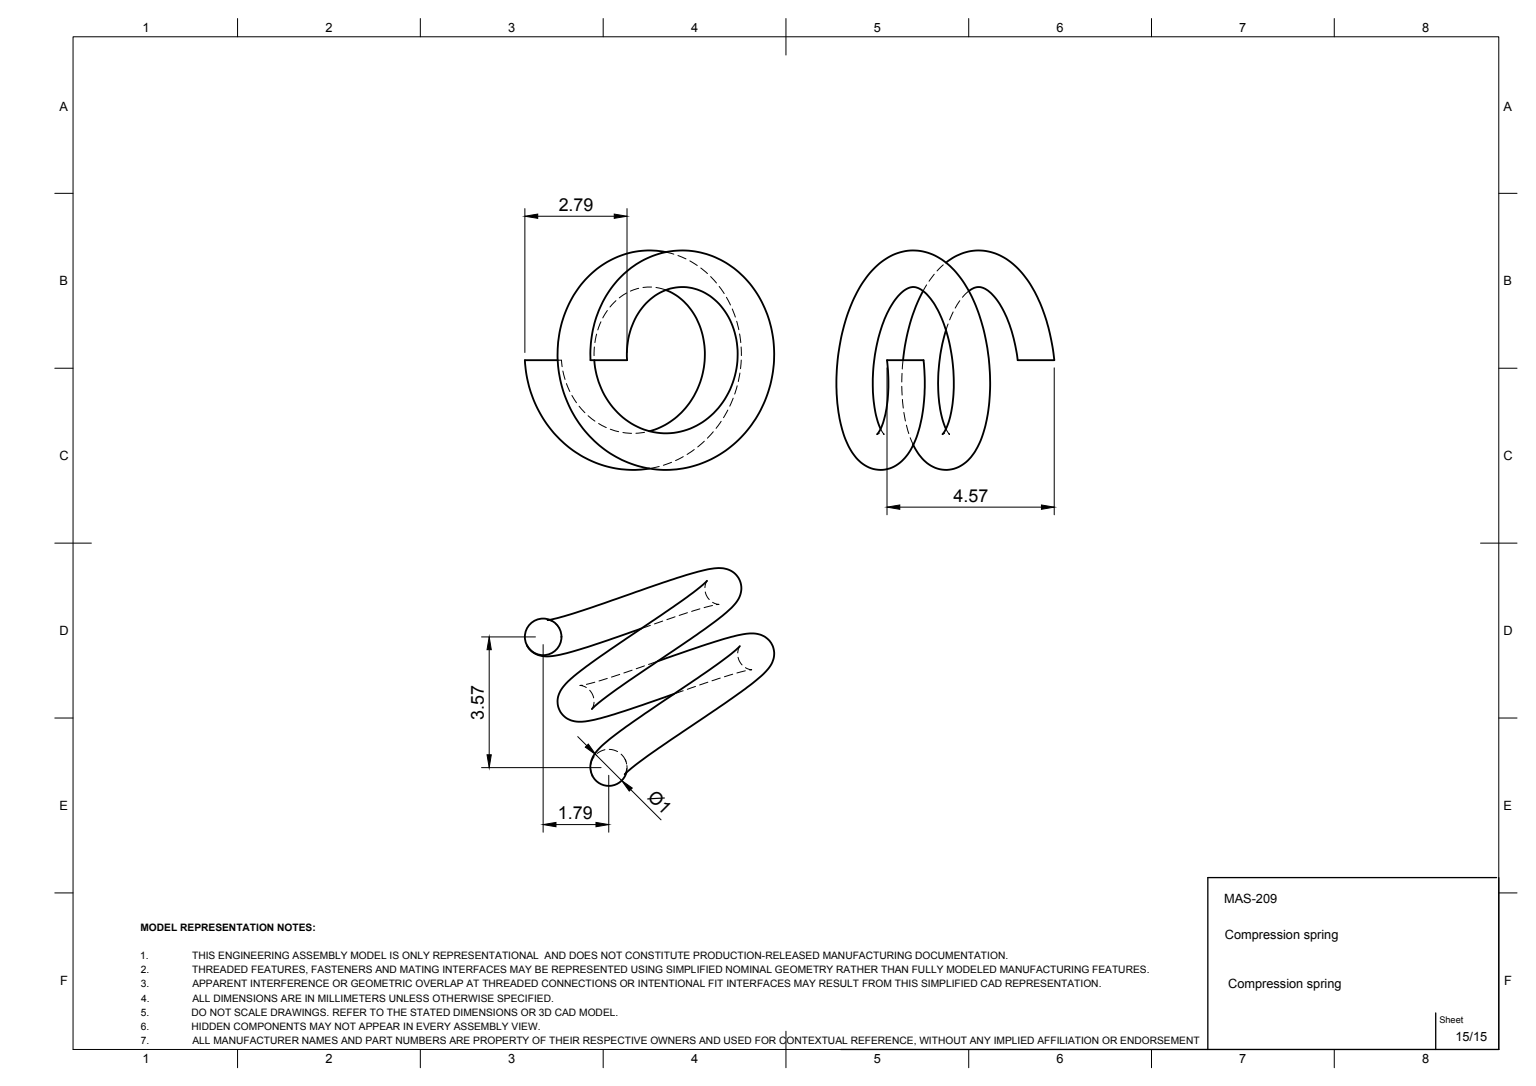
ISO-10303-21;
HEADER;
/* Generated by software containing ST-Developer
 * from STEP Tools, Inc. (www.steptools.com) 
 */

FILE_DESCRIPTION(
/* description */ ('Independent bearing-supported roller-ramp one-way clutch. Six logarit
hmic ramps with plain solid rollers, sprung guided plungers, native Co
il variants, removable shared keepers, rounded parallel key, shaft wit
h complete retaining lips, bronze journal/thrust support and bolted co
vers. Native rotor, roller planar/spin and plunger joints permit manua
l geometric engaged/released inspection. Automatic frictional torque s
witching/contact dynamics are not simulated; no capacity, hardness, fi
t, lubrication, speed, force or life rating. External input driver/cou
pling/anchors outside assembly.'),
/* implementation_level */ '2;1');

FILE_NAME(
/* name */ 'Compression spring.step',
/* time_stamp */ '2026-11-08T07:04:38-08:00',
/* author */ (''),
/* organization */ (''),
/* preprocessor_version */ 'ST-DEVELOPER v20.2',
/* originating_system */ 'Autodesk Translation Framework v15.17.0.0',
/* authorisation */ '');

FILE_SCHEMA (('AUTOMOTIVE_DESIGN { 1 0 10303 214 3 1 1 }'));
ENDSEC;

DATA;
#10=MECHANICAL_DESIGN_GEOMETRIC_PRESENTATION_REPRESENTATION('',(#313),#99526);
#281=SHAPE_REPRESENTATION_RELATIONSHIP('SRR','None',#99638,#297);
#297=ADVANCED_BREP_SHAPE_REPRESENTATION('',(#329),#99523);
#313=STYLED_ITEM('',(#99724),#329);
#329=MANIFOLD_SOLID_BREP('Body1',#18283);
#592=PLANE('',#19645);
#593=PLANE('',#19646);
#670=B_SPLINE_SURFACE_WITH_KNOTS('',3,3,((#94938,#94939,#94940,#94941,#94942,
#94943,#94944,#94945,#94946,#94947,#94948,#94949,#94950,#94951,#94952,#94953,
#94954,#94955,#94956,#94957,#94958,#94959,#94960,#94961,#94962,#94963,#94964,
#94965,#94966),(#94967,#94968,#94969,#94970,#94971,#94972,#94973,#94974,
#94975,#94976,#94977,#94978,#94979,#94980,#94981,#94982,#94983,#94984,#94985,
#94986,#94987,#94988,#94989,#94990,#94991,#94992,#94993,#94994,#94995),
(#94996,#94997,#94998,#94999,#95000,#95001,#95002,#95003,#95004,#95005,
#95006,#95007,#95008,#95009,#95010,#95011,#95012,#95013,#95014,#95015,#95016,
#95017,#95018,#95019,#95020,#95021,#95022,#95023,#95024),(#95025,#95026,
#95027,#95028,#95029,#95030,#95031,#95032,#95033,#95034,#95035,#95036,#95037,
#95038,#95039,#95040,#95041,#95042,#95043,#95044,#95045,#95046,#95047,#95048,
#95049,#95050,#95051,#95052,#95053),(#95054,#95055,#95056,#95057,#95058,
#95059,#95060,#95061,#95062,#95063,#95064,#95065,#95066,#95067,#95068,#95069,
#95070,#95071,#95072,#95073,#95074,#95075,#95076,#95077,#95078,#95079,#95080,
#95081,#95082),(#95083,#95084,#95085,#95086,#95087,#95088,#95089,#95090,
#95091,#95092,#95093,#95094,#95095,#95096,#95097,#95098,#95099,#95100,#95101,
#95102,#95103,#95104,#95105,#95106,#95107,#95108,#95109,#95110,#95111),
(#95112,#95113,#95114,#95115,#95116,#95117,#95118,#95119,#95120,#95121,
#95122,#95123,#95124,#95125,#95126,#95127,#95128,#95129,#95130,#95131,#95132,
#95133,#95134,#95135,#95136,#95137,#95138,#95139,#95140),(#95141,#95142,
#95143,#95144,#95145,#95146,#95147,#95148,#95149,#95150,#95151,#95152,#95153,
#95154,#95155,#95156,#95157,#95158,#95159,#95160,#95161,#95162,#95163,#95164,
#95165,#95166,#95167,#95168,#95169),(#95170,#95171,#95172,#95173,#95174,
#95175,#95176,#95177,#95178,#95179,#95180,#95181,#95182,#95183,#95184,#95185,
#95186,#95187,#95188,#95189,#95190,#95191,#95192,#95193,#95194,#95195,#95196,
#95197,#95198),(#95199,#95200,#95201,#95202,#95203,#95204,#95205,#95206,
#95207,#95208,#95209,#95210,#95211,#95212,#95213,#95214,#95215,#95216,#95217,
#95218,#95219,#95220,#95221,#95222,#95223,#95224,#95225,#95226,#95227)),
 .UNSPECIFIED.,.T.,.F.,.F.,(4,1,1,1,1,1,1,4),(4,1,1,1,1,1,1,1,1,1,1,1,1,
1,1,1,1,1,1,1,1,1,1,1,1,1,4),(-3.14159265358979,-2.24399475256414,-1.34639685153848,
-0.448798950512828,0.448798950512828,1.34639685153848,2.24399475256414,
3.14159265358979),(0.,0.483321946706122,0.966643893412244,1.44996584011837,
1.93328778682449,2.41660973353061,2.89993168023673,3.38325362694285,3.86657557364898,
4.3498975203551,4.83321946706122,5.31654141376734,5.79986336047346,6.28318530717959,
6.76650725388571,7.24982920059183,7.73315114729795,8.21647309400407,8.6997950407102,
9.18311698741632,9.66643893412244,10.1497608808286,10.6330828275347,11.1164047742408,
11.5997267209469,12.083048667653,12.5663706143592),.UNSPECIFIED.);
#1589=FACE_OUTER_BOUND('',#2691,.T.);
#1590=FACE_OUTER_BOUND('',#2692,.T.);
#1591=FACE_OUTER_BOUND('',#2693,.T.);
#2691=EDGE_LOOP('',(#16092,#16093,#16094,#16095));
#2692=EDGE_LOOP('',(#16096));
#2693=EDGE_LOOP('',(#16097));
#3096=CIRCLE('',#19643,0.5);
#3097=CIRCLE('',#19644,0.5);
#4515=B_SPLINE_CURVE_WITH_KNOTS('',3,(#95231,#95232,#95233,#95234,#95235,
#95236,#95237,#95238,#95239,#95240,#95241,#95242,#95243,#95244,#95245,#95246,
#95247,#95248,#95249,#95250,#95251,#95252,#95253,#95254,#95255,#95256,#95257,
#95258,#95259),.UNSPECIFIED.,.F.,.F.,(4,1,1,1,1,1,1,1,1,1,1,1,1,1,1,1,1,
1,1,1,1,1,1,1,1,1,4),(0.,0.483321946706122,0.966643893412244,1.44996584011837,
1.93328778682449,2.41660973353061,2.89993168023673,3.38325362694285,3.86657557364898,
4.3498975203551,4.83321946706122,5.31654141376734,5.79986336047346,6.28318530717959,
6.76650725388571,7.24982920059183,7.73315114729795,8.21647309400407,8.6997950407102,
9.18311698741632,9.66643893412244,10.1497608808286,10.6330828275347,11.1164047742408,
11.5997267209469,12.083048667653,12.5663706143592),.UNSPECIFIED.);
#8115=VERTEX_POINT('',#95228);
#8116=VERTEX_POINT('',#95230);
#10798=EDGE_CURVE('',#8115,#8115,#3096,.T.);
#10799=EDGE_CURVE('',#8115,#8116,#4515,.T.);
#10800=EDGE_CURVE('',#8116,#8116,#3097,.T.);
#16092=ORIENTED_EDGE('',*,*,#10798,.T.);
#16093=ORIENTED_EDGE('',*,*,#10799,.T.);
#16094=ORIENTED_EDGE('',*,*,#10800,.F.);
#16095=ORIENTED_EDGE('',*,*,#10799,.F.);
#16096=ORIENTED_EDGE('',*,*,#10800,.T.);
#16097=ORIENTED_EDGE('',*,*,#10798,.F.);
#18187=ADVANCED_FACE('',(#1589),#670,.T.);
#18188=ADVANCED_FACE('',(#1590),#592,.F.);
#18189=ADVANCED_FACE('',(#1591),#593,.T.);
#18283=CLOSED_SHELL('',(#18187,#18188,#18189));
#19642=AXIS2_PLACEMENT_3D('',#94937,#22973,#22974);
#19643=AXIS2_PLACEMENT_3D('',#95229,#22975,#22976);
#19644=AXIS2_PLACEMENT_3D('',#95260,#22977,#22978);
#19645=AXIS2_PLACEMENT_3D('',#95261,#22979,#22980);
#19646=AXIS2_PLACEMENT_3D('',#95262,#22981,#22982);
#22973=DIRECTION('axis',(0.,0.,1.));
#22974=DIRECTION('refdir',(1.,0.,0.));
#22975=DIRECTION('center_axis',(0.,0.,-1.));
#22976=DIRECTION('ref_axis',(-1.,0.,0.));
#22977=DIRECTION('center_axis',(4.89858719658941E-16,0.,-1.));
#22978=DIRECTION('ref_axis',(-1.,0.,-4.89858719658941E-16));
#22979=DIRECTION('center_axis',(-4.89858719658941E-16,0.,1.));
#22980=DIRECTION('ref_axis',(1.,0.,4.89858719658941E-16));
#22981=DIRECTION('center_axis',(0.,0.,1.));
#22982=DIRECTION('ref_axis',(1.,0.,0.));
#94937=CARTESIAN_POINT('',(0.,0.,0.));
#94938=CARTESIAN_POINT('Ctrl Pts',(3.,-6.12323399573676E-17,0.));
#94939=CARTESIAN_POINT('Ctrl Pts',(3.,0.0512820512820512,-0.483321946706122));
#94940=CARTESIAN_POINT('Ctrl Pts',(2.76209532949166,0.153846153846154,-1.44946426164245));
#94941=CARTESIAN_POINT('Ctrl Pts',(1.77197968324867,0.307692307692308,-2.56735208320081));
#94942=CARTESIAN_POINT('Ctrl Pts',(0.376021898059208,0.461538461538461,
-3.09643080035079));
#94943=CARTESIAN_POINT('Ctrl Pts',(-1.10621475336255,0.615384615384616,
-2.91679593290564));
#94944=CARTESIAN_POINT('Ctrl Pts',(-2.33474201794243,0.769230769230768,
-2.0684045486807));
#94945=CARTESIAN_POINT('Ctrl Pts',(-3.02885773675456,0.923076923076924,
-0.746548640155209));
#94946=CARTESIAN_POINT('Ctrl Pts',(-3.02855730304457,1.07692307692308,0.746474906977016));
#94947=CARTESIAN_POINT('Ctrl Pts',(-2.33497949559777,1.23076923076923,2.06860866176523));
#94948=CARTESIAN_POINT('Ctrl Pts',(-1.10608225550105,1.38461538461538,2.91650190270812));
#94949=CARTESIAN_POINT('Ctrl Pts',(0.376013421364463,1.53846153846154,3.0967529299689));
#94950=CARTESIAN_POINT('Ctrl Pts',(1.77190704246167,1.69230769230769,2.56705030189252));
#94951=CARTESIAN_POINT('Ctrl Pts',(2.76217801015642,1.84615384615384,1.44970288425454));
#94952=CARTESIAN_POINT('Ctrl Pts',(3.1191987918465,2.,1.70719823792917E-15));
#94953=CARTESIAN_POINT('Ctrl Pts',(2.76217801015642,2.15384615384615,-1.44970288425453));
#94954=CARTESIAN_POINT('Ctrl Pts',(1.77190704246167,2.30769230769231,-2.56705030189251));
#94955=CARTESIAN_POINT('Ctrl Pts',(0.376013421364468,2.46153846153846,-3.09675292996889));
#94956=CARTESIAN_POINT('Ctrl Pts',(-1.10608225550105,2.61538461538461,-2.91650190270813));
#94957=CARTESIAN_POINT('Ctrl Pts',(-2.33497949559777,2.76923076923077,-2.06860866176523));
#94958=CARTESIAN_POINT('Ctrl Pts',(-3.02855730304457,2.92307692307692,-0.746474906977022));
#94959=CARTESIAN_POINT('Ctrl Pts',(-3.02885773675456,3.07692307692307,0.746548640155207));
#94960=CARTESIAN_POINT('Ctrl Pts',(-2.33474201794243,3.23076923076923,2.0684045486807));
#94961=CARTESIAN_POINT('Ctrl Pts',(-1.10621475336255,3.38461538461538,2.91679593290564));
#94962=CARTESIAN_POINT('Ctrl Pts',(0.376021898059204,3.53846153846154,3.09643080035079));
#94963=CARTESIAN_POINT('Ctrl Pts',(1.77197968324866,3.69230769230769,2.56735208320081));
#94964=CARTESIAN_POINT('Ctrl Pts',(2.76209532949166,3.84615384615385,1.44946426164245));
#94965=CARTESIAN_POINT('Ctrl Pts',(3.,3.94871794871795,0.483321946706125));
#94966=CARTESIAN_POINT('Ctrl Pts',(3.,4.,1.46957615897682E-15));
#94967=CARTESIAN_POINT('Ctrl Pts',(3.,-0.149599650170943,0.));
#94968=CARTESIAN_POINT('Ctrl Pts',(3.,-0.0983175988888913,-0.4835411540332));
#94969=CARTESIAN_POINT('Ctrl Pts',(2.76209576921471,0.00424650367521139,
-1.44932835794453));
#94970=CARTESIAN_POINT('Ctrl Pts',(1.77200161890609,0.158092657521365,-2.56746394660749));
#94971=CARTESIAN_POINT('Ctrl Pts',(0.376023954420967,0.311938811367519,
-3.09638050731302));
#94972=CARTESIAN_POINT('Ctrl Pts',(-1.10623737843825,0.465784965213672,
-2.91686578526799));
#94973=CARTESIAN_POINT('Ctrl Pts',(-2.33472522086381,0.619631119059827,
-2.06838287160141));
#94974=CARTESIAN_POINT('Ctrl Pts',(-3.02891313603334,0.77347727290598,-0.746566701745084));
#94975=CARTESIAN_POINT('Ctrl Pts',(-3.02853676566909,0.927323426752134,
0.746472023741791));
#94976=CARTESIAN_POINT('Ctrl Pts',(-2.33502184745744,1.08116958059829,2.0686447945416));
#94977=CARTESIAN_POINT('Ctrl Pts',(-1.10607478639173,1.23501573444444,2.91648299449822));
#94978=CARTESIAN_POINT('Ctrl Pts',(0.376020159868782,1.3888618882906,3.09680852875374));
#94979=CARTESIAN_POINT('Ctrl Pts',(1.77189524100041,1.54270804213675,2.56703330753083));
#94980=CARTESIAN_POINT('Ctrl Pts',(2.76222787027974,1.6965541959829,1.44972899802138));
#94981=CARTESIAN_POINT('Ctrl Pts',(3.1191779858324,1.85040034982906,1.3413700440872E-15));
#94982=CARTESIAN_POINT('Ctrl Pts',(2.76222787027974,2.00424650367521,-1.44972899802137));
#94983=CARTESIAN_POINT('Ctrl Pts',(1.77189524100041,2.15809265752137,-2.56703330753083));
#94984=CARTESIAN_POINT('Ctrl Pts',(0.376020159868788,2.31193881136752,-3.09680852875374));
#94985=CARTESIAN_POINT('Ctrl Pts',(-1.10607478639173,2.46578496521367,-2.91648299449822));
#94986=CARTESIAN_POINT('Ctrl Pts',(-2.33502184745743,2.61963111905983,-2.0686447945416));
#94987=CARTESIAN_POINT('Ctrl Pts',(-3.0285367656691,2.77347727290598,-0.746472023741798));
#94988=CARTESIAN_POINT('Ctrl Pts',(-3.02891313603333,2.92732342675214,0.746566701745082));
#94989=CARTESIAN_POINT('Ctrl Pts',(-2.33472522086383,3.08116958059829,2.06838287160141));
#94990=CARTESIAN_POINT('Ctrl Pts',(-1.10623737843825,3.23501573444444,2.91686578526799));
#94991=CARTESIAN_POINT('Ctrl Pts',(0.376023954420961,3.38886188829059,3.09638050731302));
#94992=CARTESIAN_POINT('Ctrl Pts',(1.77200161890609,3.54270804213675,2.56746394660749));
#94993=CARTESIAN_POINT('Ctrl Pts',(2.76209576921471,3.69655419598291,1.44932835794453));
#94994=CARTESIAN_POINT('Ctrl Pts',(3.,3.79911829854701,0.483541154033203));
#94995=CARTESIAN_POINT('Ctrl Pts',(3.,3.85040034982906,1.46957615897682E-15));
#94996=CARTESIAN_POINT('Ctrl Pts',(2.85712660496334,-0.447398096836595,
0.));
#94997=CARTESIAN_POINT('Ctrl Pts',(2.85712660496334,-0.396116045554544,
-0.460194067158232));
#94998=CARTESIAN_POINT('Ctrl Pts',(2.63055179659491,-0.293551942990442,
-1.38050245605029));
#94999=CARTESIAN_POINT('Ctrl Pts',(1.68757909829609,-0.139705789144288,
-2.44502721529682));
#95000=CARTESIAN_POINT('Ctrl Pts',(0.358113025085229,0.0141403647018659,
-2.94899016152089));
#95001=CARTESIAN_POINT('Ctrl Pts',(-1.05352052128293,0.16798651854802,-2.77785005675019));
#95002=CARTESIAN_POINT('Ctrl Pts',(-2.22355960197289,0.321832672394174,
-1.96990875947179));
#95003=CARTESIAN_POINT('Ctrl Pts',(-2.88458222522762,0.475678826240328,
-0.710985602845217));
#95004=CARTESIAN_POINT('Ctrl Pts',(-2.88433418102835,0.62952498008648,0.71092588480246));
#95005=CARTESIAN_POINT('Ctrl Pts',(-2.22375610724719,0.783371133932636,
1.97007416068242));
#95006=CARTESIAN_POINT('Ctrl Pts',(-1.05340942551119,0.937217287778789,
2.77761454217348));
#95007=CARTESIAN_POINT('Ctrl Pts',(0.358102604038195,1.09106344162494,2.94924384613783));
#95008=CARTESIAN_POINT('Ctrl Pts',(1.68752683583458,1.2449095954711,2.44480442711754));
#95009=CARTESIAN_POINT('Ctrl Pts',(2.63060575577254,1.39875574931725,1.38064846415744));
#95010=CARTESIAN_POINT('Ctrl Pts',(2.97065905213792,1.5526019031634,-2.4388546256131E-16));
#95011=CARTESIAN_POINT('Ctrl Pts',(2.63060575577254,1.70644805700956,-1.38064846415743));
#95012=CARTESIAN_POINT('Ctrl Pts',(1.68752683583459,1.86029421085571,-2.44480442711754));
#95013=CARTESIAN_POINT('Ctrl Pts',(0.358102604038199,2.01414036470186,-2.94924384613782));
#95014=CARTESIAN_POINT('Ctrl Pts',(-1.05340942551119,2.16798651854802,-2.77761454217349));
#95015=CARTESIAN_POINT('Ctrl Pts',(-2.22375610724719,2.32183267239418,-1.97007416068241));
#95016=CARTESIAN_POINT('Ctrl Pts',(-2.88433418102835,2.47567882624033,-0.710925884802468));
#95017=CARTESIAN_POINT('Ctrl Pts',(-2.88458222522762,2.62952498008648,0.710985602845219));
#95018=CARTESIAN_POINT('Ctrl Pts',(-2.2235596019729,2.78337113393263,1.96990875947178));
#95019=CARTESIAN_POINT('Ctrl Pts',(-1.05352052128293,2.93721728777879,2.7778500567502));
#95020=CARTESIAN_POINT('Ctrl Pts',(0.358113025085224,3.09106344162494,2.94899016152089));
#95021=CARTESIAN_POINT('Ctrl Pts',(1.68757909829608,3.2449095954711,2.44502721529682));
#95022=CARTESIAN_POINT('Ctrl Pts',(2.63055179659491,3.39875574931725,1.3805024560503));
#95023=CARTESIAN_POINT('Ctrl Pts',(2.85712660496334,3.50131985188135,0.460194067158235));
#95024=CARTESIAN_POINT('Ctrl Pts',(2.85712660496334,3.55260190316341,1.39958838061084E-15));
#95025=CARTESIAN_POINT('Ctrl Pts',(2.3726759939225,-0.557941290809918,0.));
#95026=CARTESIAN_POINT('Ctrl Pts',(2.3726759939225,-0.506659239527867,-0.382282398128741));
#95027=CARTESIAN_POINT('Ctrl Pts',(2.18451914777363,-0.404095136963764,
-1.14635298489711));
#95028=CARTESIAN_POINT('Ctrl Pts',(1.40144724769161,-0.25024898311761,-2.03051196529879));
#95029=CARTESIAN_POINT('Ctrl Pts',(0.297392962941051,-0.0964028292714561,
-2.44893616184819));
#95030=CARTESIAN_POINT('Ctrl Pts',(-0.874899176834334,0.0574433245746974,
-2.3068791471024));
#95031=CARTESIAN_POINT('Ctrl Pts',(-1.84652671515893,0.211289478420851,
-1.63588194226376));
#95032=CARTESIAN_POINT('Ctrl Pts',(-2.39550615492902,0.365135632267005,
-0.590441565156793));
#95033=CARTESIAN_POINT('Ctrl Pts',(-2.39525921257935,0.518981786113159,
0.590380676300523));
#95034=CARTESIAN_POINT('Ctrl Pts',(-1.84672180305351,0.672827939959313,
1.63605047782857));
#95035=CARTESIAN_POINT('Ctrl Pts',(-0.874790687110246,0.826674093805466,
2.30663569332898));
#95036=CARTESIAN_POINT('Ctrl Pts',(0.297386834171931,0.98052024765162,2.44920394446013));
#95037=CARTESIAN_POINT('Ctrl Pts',(1.40138565077454,1.13436640149777,2.03025745375436));
#95038=CARTESIAN_POINT('Ctrl Pts',(2.18459061244276,1.28821255534393,1.14656161967552));
#95039=CARTESIAN_POINT('Ctrl Pts',(2.4669468077447,1.44205870919008,2.4388546256131E-16));
#95040=CARTESIAN_POINT('Ctrl Pts',(2.18459061244276,1.59590486303624,-1.14656161967552));
#95041=CARTESIAN_POINT('Ctrl Pts',(1.40138565077454,1.74975101688239,-2.03025745375436));
#95042=CARTESIAN_POINT('Ctrl Pts',(0.297386834171934,1.90359717072855,-2.44920394446012));
#95043=CARTESIAN_POINT('Ctrl Pts',(-0.874790687110244,2.0574433245747,-2.30663569332898));
#95044=CARTESIAN_POINT('Ctrl Pts',(-1.84672180305351,2.21128947842085,-1.63605047782857));
#95045=CARTESIAN_POINT('Ctrl Pts',(-2.39525921257935,2.36513563226701,-0.590380676300528));
#95046=CARTESIAN_POINT('Ctrl Pts',(-2.39550615492902,2.51898178611316,0.590441565156791));
#95047=CARTESIAN_POINT('Ctrl Pts',(-1.84652671515893,2.67282793995932,1.63588194226375));
#95048=CARTESIAN_POINT('Ctrl Pts',(-0.874899176834338,2.82667409380547,
2.3068791471024));
#95049=CARTESIAN_POINT('Ctrl Pts',(0.29739296294105,2.98052024765162,2.4489361618482));
#95050=CARTESIAN_POINT('Ctrl Pts',(1.4014472476916,3.13436640149777,2.03051196529879));
#95051=CARTESIAN_POINT('Ctrl Pts',(2.18451914777363,3.28821255534393,1.14635298489712));
#95052=CARTESIAN_POINT('Ctrl Pts',(2.3726759939225,3.39077665790803,0.382282398128744));
#95053=CARTESIAN_POINT('Ctrl Pts',(2.3726759939225,3.44205870919008,1.16227602454838E-15));
#95054=CARTESIAN_POINT('Ctrl Pts',(1.98402625071561,-0.248351324860585,
0.));
#95055=CARTESIAN_POINT('Ctrl Pts',(1.98402625071561,-0.197069273578533,
-0.319662635491883));
#95056=CARTESIAN_POINT('Ctrl Pts',(1.82668992334287,-0.0945051710144311,
-0.958578390155419));
#95057=CARTESIAN_POINT('Ctrl Pts',(1.17188688645211,0.059340982831723,-1.69790894363414));
#95058=CARTESIAN_POINT('Ctrl Pts',(0.248679307147478,0.213187136677876,
-2.0477950661503));
#95059=CARTESIAN_POINT('Ctrl Pts',(-0.731588588146289,0.367033290524031,
-1.92900674830902));
#95060=CARTESIAN_POINT('Ctrl Pts',(-1.54406150387629,0.520879444370184,
-1.36792084856094));
#95061=CARTESIAN_POINT('Ctrl Pts',(-2.00311651810014,0.674725598216338,
-0.493725804019771));
#95062=CARTESIAN_POINT('Ctrl Pts',(-2.00291038342168,0.82857175206249,0.493674987626987));
#95063=CARTESIAN_POINT('Ctrl Pts',(-1.54422435711181,0.982417905908647,
1.3680615051111));
#95064=CARTESIAN_POINT('Ctrl Pts',(-0.731498011144787,1.1362640597548,1.92880359121951));
#95065=CARTESIAN_POINT('Ctrl Pts',(0.248674160214009,1.29011021360096,2.04801848620564));
#95066=CARTESIAN_POINT('Ctrl Pts',(1.17183553828091,1.44395636744711,1.69769672907218));
#95067=CARTESIAN_POINT('Ctrl Pts',(1.82674944897787,1.59780252129326,0.958752086361943));
#95068=CARTESIAN_POINT('Ctrl Pts',(2.06285538814528,1.75164867513941,8.53599118964584E-16));
#95069=CARTESIAN_POINT('Ctrl Pts',(1.82674944897787,1.90549482898556,-0.958752086361939));
#95070=CARTESIAN_POINT('Ctrl Pts',(1.17183553828091,2.05934098283173,-1.69769672907218));
#95071=CARTESIAN_POINT('Ctrl Pts',(0.248674160214013,2.21318713667787,-2.04801848620563));
#95072=CARTESIAN_POINT('Ctrl Pts',(-0.731498011144785,2.36703329052403,
-1.92880359121952));
#95073=CARTESIAN_POINT('Ctrl Pts',(-1.54422435711181,2.52087944437019,-1.36806150511109));
#95074=CARTESIAN_POINT('Ctrl Pts',(-2.00291038342167,2.67472559821633,-0.493674987626991));
#95075=CARTESIAN_POINT('Ctrl Pts',(-2.00311651810014,2.8285717520625,0.49372580401977));
#95076=CARTESIAN_POINT('Ctrl Pts',(-1.54406150387629,2.98241790590864,1.36792084856094));
#95077=CARTESIAN_POINT('Ctrl Pts',(-0.731588588146291,3.1362640597548,1.92900674830902));
#95078=CARTESIAN_POINT('Ctrl Pts',(0.248679307147477,3.29011021360095,2.0477950661503));
#95079=CARTESIAN_POINT('Ctrl Pts',(1.17188688645211,3.44395636744711,1.69790894363414));
#95080=CARTESIAN_POINT('Ctrl Pts',(1.82668992334286,3.59780252129326,0.958578390155423));
#95081=CARTESIAN_POINT('Ctrl Pts',(1.9840262507156,3.70036662385736,0.319662635491885));
#95082=CARTESIAN_POINT('Ctrl Pts',(1.98402625071561,3.75164867513941,9.71892558945275E-16));
#95083=CARTESIAN_POINT('Ctrl Pts',(1.98458281684753,0.248133119200085,0.));
#95084=CARTESIAN_POINT('Ctrl Pts',(1.98458281684753,0.299415170482137,-0.319687116399019));
#95085=CARTESIAN_POINT('Ctrl Pts',(1.82720222215302,0.401979273046239,-0.958887711587539));
#95086=CARTESIAN_POINT('Ctrl Pts',(1.17220910470982,0.555825426892393,-1.69835197907329));
#95087=CARTESIAN_POINT('Ctrl Pts',(0.24874845599561,0.709671580738547,-2.04838447802754));
#95088=CARTESIAN_POINT('Ctrl Pts',(-0.731787087320181,0.863517734584699,
-1.92952710616438));
#95089=CARTESIAN_POINT('Ctrl Pts',(-1.54449964495675,1.01736388843086,-1.36831102934188));
#95090=CARTESIAN_POINT('Ctrl Pts',(-2.0036619638227,1.17121004227701,-0.493858934250917));
#95091=CARTESIAN_POINT('Ctrl Pts',(-2.00347835478891,1.32505619612316,0.493814332568918));
#95092=CARTESIAN_POINT('Ctrl Pts',(-1.54464495305281,1.47890234996932,1.36843453276745));
#95093=CARTESIAN_POINT('Ctrl Pts',(-0.731705434884396,1.63274850381547,
1.92935028937276));
#95094=CARTESIAN_POINT('Ctrl Pts',(0.2487419151547,1.78659465766162,2.04857646865583));
#95095=CARTESIAN_POINT('Ctrl Pts',(1.17216777551306,1.94044081150778,1.69817802712664));
#95096=CARTESIAN_POINT('Ctrl Pts',(1.82724706691833,2.09428696535393,0.959013272719332));
#95097=CARTESIAN_POINT('Ctrl Pts',(2.06344025539221,2.24813311920008,1.58525550664851E-15));
#95098=CARTESIAN_POINT('Ctrl Pts',(1.82724706691833,2.40197927304624,-0.959013272719332));
#95099=CARTESIAN_POINT('Ctrl Pts',(1.17216777551307,2.55582542689239,-1.69817802712664));
#95100=CARTESIAN_POINT('Ctrl Pts',(0.248741915154701,2.70967158073855,-2.04857646865583));
#95101=CARTESIAN_POINT('Ctrl Pts',(-0.731705434884394,2.8635177345847,-1.92935028937276));
#95102=CARTESIAN_POINT('Ctrl Pts',(-1.54464495305281,3.01736388843085,-1.36843453276745));
#95103=CARTESIAN_POINT('Ctrl Pts',(-2.00347835478892,3.17121004227701,-0.493814332568922));
#95104=CARTESIAN_POINT('Ctrl Pts',(-2.0036619638227,3.32505619612316,0.493858934250916));
#95105=CARTESIAN_POINT('Ctrl Pts',(-1.54449964495675,3.47890234996932,1.36831102934188));
#95106=CARTESIAN_POINT('Ctrl Pts',(-0.731787087320183,3.63274850381547,
1.92952710616438));
#95107=CARTESIAN_POINT('Ctrl Pts',(0.248748455995608,3.78659465766163,2.04838447802754));
#95108=CARTESIAN_POINT('Ctrl Pts',(1.17220910470981,3.94044081150777,1.69835197907329));
#95109=CARTESIAN_POINT('Ctrl Pts',(1.82720222215303,4.09428696535394,0.95888771158754));
#95110=CARTESIAN_POINT('Ctrl Pts',(1.98458281684753,4.19685106791804,0.319687116399021));
#95111=CARTESIAN_POINT('Ctrl Pts',(1.98458281684753,4.24813311920009,9.72165197718065E-16));
#95112=CARTESIAN_POINT('Ctrl Pts',(2.37244316231612,0.558475305697687,0.));
#95113=CARTESIAN_POINT('Ctrl Pts',(2.37244316231612,0.609757356979738,-0.382293167894848));
#95114=CARTESIAN_POINT('Ctrl Pts',(2.18430487692558,0.712321459543841,-1.14621055826918));
#95115=CARTESIAN_POINT('Ctrl Pts',(1.40131455475087,0.866167613389996,-2.03033734976027));
#95116=CARTESIAN_POINT('Ctrl Pts',(0.297364232596012,1.02001376723615,-2.44868476910202));
#95117=CARTESIAN_POINT('Ctrl Pts',(-0.874818306111391,1.1738599210823,-2.3066681580635));
#95118=CARTESIAN_POINT('Ctrl Pts',(-1.84634181500677,1.32770607492845,-1.63571663787998));
#95119=CARTESIAN_POINT('Ctrl Pts',(-2.39528328540685,1.48155222877461,-0.590387603200993));
#95120=CARTESIAN_POINT('Ctrl Pts',(-2.39501964124714,1.63539838262076,0.590322106947738));
#95121=CARTESIAN_POINT('Ctrl Pts',(-1.8465499120856,1.78924453646692,1.63589789028415));
#95122=CARTESIAN_POINT('Ctrl Pts',(-0.874703198395058,1.94309069031307,
2.3064051775018));
#95123=CARTESIAN_POINT('Ctrl Pts',(0.297359135731523,2.09693684415923,2.44897584949709));
#95124=CARTESIAN_POINT('Ctrl Pts',(1.40124553283611,2.25078299800538,2.03005448058009));
#95125=CARTESIAN_POINT('Ctrl Pts',(2.18438722007224,2.40462915185154,1.14645485904265));
#95126=CARTESIAN_POINT('Ctrl Pts',(2.46670014251008,2.55847530569768,1.58525550664851E-15));
#95127=CARTESIAN_POINT('Ctrl Pts',(2.18438722007224,2.71232145954384,-1.14645485904265));
#95128=CARTESIAN_POINT('Ctrl Pts',(1.40124553283611,2.86616761338999,-2.03005448058009));
#95129=CARTESIAN_POINT('Ctrl Pts',(0.297359135731528,3.02001376723615,-2.44897584949709));
#95130=CARTESIAN_POINT('Ctrl Pts',(-0.874703198395057,3.1738599210823,-2.3064051775018));
#95131=CARTESIAN_POINT('Ctrl Pts',(-1.84654991208559,3.32770607492846,-1.63589789028415));
#95132=CARTESIAN_POINT('Ctrl Pts',(-2.39501964124714,3.48155222877461,-0.590322106947741));
#95133=CARTESIAN_POINT('Ctrl Pts',(-2.39528328540685,3.63539838262076,0.590387603200988));
#95134=CARTESIAN_POINT('Ctrl Pts',(-1.84634181500678,3.78924453646692,1.63571663787998));
#95135=CARTESIAN_POINT('Ctrl Pts',(-0.874818306111389,3.94309069031306,
2.30666815806349));
#95136=CARTESIAN_POINT('Ctrl Pts',(0.297364232596008,4.09693684415923,2.44868476910202));
#95137=CARTESIAN_POINT('Ctrl Pts',(1.40131455475086,4.25078299800537,2.03033734976027));
#95138=CARTESIAN_POINT('Ctrl Pts',(2.18430487692558,4.40462915185153,1.14621055826919));
#95139=CARTESIAN_POINT('Ctrl Pts',(2.37244316231612,4.50719325441563,0.38229316789485));
#95140=CARTESIAN_POINT('Ctrl Pts',(2.37244316231612,4.55847530569768,1.16216196995579E-15));
#95141=CARTESIAN_POINT('Ctrl Pts',(2.85700819365424,0.447072546346698,0.));
#95142=CARTESIAN_POINT('Ctrl Pts',(2.85700819365424,0.49835459762875,-0.460152253076002));
#95143=CARTESIAN_POINT('Ctrl Pts',(2.63044272987694,0.600918700192852,-1.38045934159639));
#95144=CARTESIAN_POINT('Ctrl Pts',(1.68750688222128,0.754764854039006,-2.44491427782217));
#95145=CARTESIAN_POINT('Ctrl Pts',(0.358097970041885,0.90861100788516,-2.94887316066247));
#95146=CARTESIAN_POINT('Ctrl Pts',(-1.05347451173092,1.06245716173131,-2.77772768414576));
#95147=CARTESIAN_POINT('Ctrl Pts',(-2.22346919095397,1.21630331557747,-1.96982936708426));
#95148=CARTESIAN_POINT('Ctrl Pts',(-2.88445692863269,1.37014946942362,-0.710954262816585));
#95149=CARTESIAN_POINT('Ctrl Pts',(-2.8842167727775,1.52399562326978,0.710896720174062));
#95150=CARTESIAN_POINT('Ctrl Pts',(-2.22365955166528,1.67784177711593,1.96998876394438));
#95151=CARTESIAN_POINT('Ctrl Pts',(-1.05336654269098,1.83168793096208,2.77750138781392));
#95152=CARTESIAN_POINT('Ctrl Pts',(0.358087063676883,1.98553408480824,2.94911584899633));
#95153=CARTESIAN_POINT('Ctrl Pts',(1.6874581219902,2.13938023865439,2.44470486725235));
#95154=CARTESIAN_POINT('Ctrl Pts',(2.6304915596885,2.29322639250055,1.38058853511652));
#95155=CARTESIAN_POINT('Ctrl Pts',(2.97053809409234,2.4470725463467,1.58525550664851E-15));
#95156=CARTESIAN_POINT('Ctrl Pts',(2.6304915596885,2.60091870019286,-1.38058853511652));
#95157=CARTESIAN_POINT('Ctrl Pts',(1.68745812199021,2.754764854039,-2.44470486725235));
#95158=CARTESIAN_POINT('Ctrl Pts',(0.358087063676885,2.90861100788517,-2.94911584899632));
#95159=CARTESIAN_POINT('Ctrl Pts',(-1.05336654269097,3.06245716173131,-2.77750138781392));
#95160=CARTESIAN_POINT('Ctrl Pts',(-2.22365955166528,3.21630331557747,-1.96998876394438));
#95161=CARTESIAN_POINT('Ctrl Pts',(-2.8842167727775,3.37014946942362,-0.710896720174069));
#95162=CARTESIAN_POINT('Ctrl Pts',(-2.88445692863269,3.52399562326977,0.710954262816585));
#95163=CARTESIAN_POINT('Ctrl Pts',(-2.22346919095397,3.67784177711593,1.96982936708426));
#95164=CARTESIAN_POINT('Ctrl Pts',(-1.05347451173092,3.83168793096208,2.77772768414576));
#95165=CARTESIAN_POINT('Ctrl Pts',(0.358097970041882,3.98553408480824,2.94887316066247));
#95166=CARTESIAN_POINT('Ctrl Pts',(1.68750688222128,4.13938023865439,2.44491427782217));
#95167=CARTESIAN_POINT('Ctrl Pts',(2.63044272987694,4.29322639250055,1.38045934159639));
#95168=CARTESIAN_POINT('Ctrl Pts',(2.85700819365424,4.39579049506465,0.460152253076004));
#95169=CARTESIAN_POINT('Ctrl Pts',(2.85700819365424,4.44707254634671,1.39953037579857E-15));
#95170=CARTESIAN_POINT('Ctrl Pts',(3.,0.149599650170943,0.));
#95171=CARTESIAN_POINT('Ctrl Pts',(3.,0.200881701452994,-0.483569736915588));
#95172=CARTESIAN_POINT('Ctrl Pts',(2.76209582655108,0.303445804017096,-1.44931063718918));
#95173=CARTESIAN_POINT('Ctrl Pts',(1.7720044791404,0.45729195786325,-2.56747853270112));
#95174=CARTESIAN_POINT('Ctrl Pts',(0.376024222554094,0.611138111709404,
-3.0963739495031));
#95175=CARTESIAN_POINT('Ctrl Pts',(-1.10624032856718,0.764984265555557,
-2.91687489345741));
#95176=CARTESIAN_POINT('Ctrl Pts',(-2.3347230306591,0.918830419401713,-2.06838004508363));
#95177=CARTESIAN_POINT('Ctrl Pts',(-3.02892035965624,1.07267657324786,-0.746569056831962));
#95178=CARTESIAN_POINT('Ctrl Pts',(-3.02853408775958,1.22652272709402,0.746471647790977));
#95179=CARTESIAN_POINT('Ctrl Pts',(-2.33502736980124,1.38036888094017,2.06864950596667));
#95180=CARTESIAN_POINT('Ctrl Pts',(-1.10607381247961,1.53421503478633,2.91648052901886));
#95181=CARTESIAN_POINT('Ctrl Pts',(0.376021038515855,1.68806118863248,3.09681577839064));
#95182=CARTESIAN_POINT('Ctrl Pts',(1.77189370218424,1.84190734247864,2.56703109160197));
#95183=CARTESIAN_POINT('Ctrl Pts',(2.76223437164108,1.99575349632479,1.44973240304774));
#95184=CARTESIAN_POINT('Ctrl Pts',(3.11917527289456,2.14959965017094,1.3413700440872E-15));
#95185=CARTESIAN_POINT('Ctrl Pts',(2.76223437164108,2.3034458040171,-1.44973240304773));
#95186=CARTESIAN_POINT('Ctrl Pts',(1.77189370218425,2.45729195786325,-2.56703109160197));
#95187=CARTESIAN_POINT('Ctrl Pts',(0.37602103851586,2.61113811170941,-3.09681577839064));
#95188=CARTESIAN_POINT('Ctrl Pts',(-1.10607381247961,2.76498426555556,-2.91648052901886));
#95189=CARTESIAN_POINT('Ctrl Pts',(-2.33502736980123,2.91883041940171,-2.06864950596667));
#95190=CARTESIAN_POINT('Ctrl Pts',(-3.02853408775958,3.07267657324787,-0.746471647790982));
#95191=CARTESIAN_POINT('Ctrl Pts',(-3.02892035965624,3.22652272709402,0.746569056831959));
#95192=CARTESIAN_POINT('Ctrl Pts',(-2.3347230306591,3.38036888094017,2.06838004508363));
#95193=CARTESIAN_POINT('Ctrl Pts',(-1.10624032856718,3.53421503478633,2.91687489345741));
#95194=CARTESIAN_POINT('Ctrl Pts',(0.376024222554089,3.68806118863248,3.09637394950311));
#95195=CARTESIAN_POINT('Ctrl Pts',(1.7720044791404,3.84190734247863,2.56747853270111));
#95196=CARTESIAN_POINT('Ctrl Pts',(2.76209582655107,3.99575349632479,1.44931063718918));
#95197=CARTESIAN_POINT('Ctrl Pts',(3.,4.09831759888889,0.483569736915591));
#95198=CARTESIAN_POINT('Ctrl Pts',(3.,4.14959965017094,1.46957615897682E-15));
#95199=CARTESIAN_POINT('Ctrl Pts',(3.,6.12323399573676E-17,0.));
#95200=CARTESIAN_POINT('Ctrl Pts',(3.,0.0512820512820513,-0.483321946706122));
#95201=CARTESIAN_POINT('Ctrl Pts',(2.76209532949166,0.153846153846154,-1.44946426164245));
#95202=CARTESIAN_POINT('Ctrl Pts',(1.77197968324867,0.307692307692308,-2.56735208320081));
#95203=CARTESIAN_POINT('Ctrl Pts',(0.376021898059208,0.461538461538461,
-3.09643080035079));
#95204=CARTESIAN_POINT('Ctrl Pts',(-1.10621475336255,0.615384615384616,
-2.91679593290564));
#95205=CARTESIAN_POINT('Ctrl Pts',(-2.33474201794243,0.769230769230768,
-2.0684045486807));
#95206=CARTESIAN_POINT('Ctrl Pts',(-3.02885773675456,0.923076923076924,
-0.746548640155209));
#95207=CARTESIAN_POINT('Ctrl Pts',(-3.02855730304457,1.07692307692308,0.746474906977016));
#95208=CARTESIAN_POINT('Ctrl Pts',(-2.33497949559777,1.23076923076923,2.06860866176523));
#95209=CARTESIAN_POINT('Ctrl Pts',(-1.10608225550105,1.38461538461539,2.91650190270812));
#95210=CARTESIAN_POINT('Ctrl Pts',(0.376013421364463,1.53846153846154,3.0967529299689));
#95211=CARTESIAN_POINT('Ctrl Pts',(1.77190704246167,1.69230769230769,2.56705030189252));
#95212=CARTESIAN_POINT('Ctrl Pts',(2.76217801015642,1.84615384615384,1.44970288425454));
#95213=CARTESIAN_POINT('Ctrl Pts',(3.1191987918465,2.,1.70719823792917E-15));
#95214=CARTESIAN_POINT('Ctrl Pts',(2.76217801015642,2.15384615384615,-1.44970288425453));
#95215=CARTESIAN_POINT('Ctrl Pts',(1.77190704246167,2.30769230769231,-2.56705030189251));
#95216=CARTESIAN_POINT('Ctrl Pts',(0.376013421364468,2.46153846153846,-3.09675292996889));
#95217=CARTESIAN_POINT('Ctrl Pts',(-1.10608225550105,2.61538461538461,-2.91650190270813));
#95218=CARTESIAN_POINT('Ctrl Pts',(-2.33497949559777,2.76923076923077,-2.06860866176523));
#95219=CARTESIAN_POINT('Ctrl Pts',(-3.02855730304457,2.92307692307692,-0.746474906977022));
#95220=CARTESIAN_POINT('Ctrl Pts',(-3.02885773675456,3.07692307692307,0.746548640155207));
#95221=CARTESIAN_POINT('Ctrl Pts',(-2.33474201794243,3.23076923076923,2.0684045486807));
#95222=CARTESIAN_POINT('Ctrl Pts',(-1.10621475336255,3.38461538461538,2.91679593290564));
#95223=CARTESIAN_POINT('Ctrl Pts',(0.376021898059204,3.53846153846154,3.09643080035079));
#95224=CARTESIAN_POINT('Ctrl Pts',(1.77197968324866,3.69230769230769,2.56735208320081));
#95225=CARTESIAN_POINT('Ctrl Pts',(2.76209532949166,3.84615384615385,1.44946426164245));
#95226=CARTESIAN_POINT('Ctrl Pts',(3.,3.94871794871795,0.483321946706125));
#95227=CARTESIAN_POINT('Ctrl Pts',(3.,4.,1.46957615897682E-15));
#95228=CARTESIAN_POINT('',(3.,-6.12323399573676E-17,0.));
#95229=CARTESIAN_POINT('Origin',(2.5,0.,0.));
#95230=CARTESIAN_POINT('',(3.,4.,1.46957615897682E-15));
#95231=CARTESIAN_POINT('Ctrl Pts',(3.,6.12323399573676E-17,0.));
#95232=CARTESIAN_POINT('Ctrl Pts',(3.,0.0512820512820513,-0.483321946706122));
#95233=CARTESIAN_POINT('Ctrl Pts',(2.76209532949166,0.153846153846154,-1.44946426164245));
#95234=CARTESIAN_POINT('Ctrl Pts',(1.77197968324867,0.307692307692308,-2.56735208320081));
#95235=CARTESIAN_POINT('Ctrl Pts',(0.376021898059208,0.461538461538461,
-3.09643080035079));
#95236=CARTESIAN_POINT('Ctrl Pts',(-1.10621475336255,0.615384615384616,
-2.91679593290564));
#95237=CARTESIAN_POINT('Ctrl Pts',(-2.33474201794243,0.769230769230768,
-2.0684045486807));
#95238=CARTESIAN_POINT('Ctrl Pts',(-3.02885773675456,0.923076923076924,
-0.746548640155209));
#95239=CARTESIAN_POINT('Ctrl Pts',(-3.02855730304457,1.07692307692308,0.746474906977016));
#95240=CARTESIAN_POINT('Ctrl Pts',(-2.33497949559777,1.23076923076923,2.06860866176523));
#95241=CARTESIAN_POINT('Ctrl Pts',(-1.10608225550105,1.38461538461539,2.91650190270812));
#95242=CARTESIAN_POINT('Ctrl Pts',(0.376013421364463,1.53846153846154,3.0967529299689));
#95243=CARTESIAN_POINT('Ctrl Pts',(1.77190704246167,1.69230769230769,2.56705030189252));
#95244=CARTESIAN_POINT('Ctrl Pts',(2.76217801015642,1.84615384615384,1.44970288425454));
#95245=CARTESIAN_POINT('Ctrl Pts',(3.1191987918465,2.,1.70719823792917E-15));
#95246=CARTESIAN_POINT('Ctrl Pts',(2.76217801015642,2.15384615384615,-1.44970288425453));
#95247=CARTESIAN_POINT('Ctrl Pts',(1.77190704246167,2.30769230769231,-2.56705030189251));
#95248=CARTESIAN_POINT('Ctrl Pts',(0.376013421364468,2.46153846153846,-3.09675292996889));
#95249=CARTESIAN_POINT('Ctrl Pts',(-1.10608225550105,2.61538461538461,-2.91650190270813));
#95250=CARTESIAN_POINT('Ctrl Pts',(-2.33497949559777,2.76923076923077,-2.06860866176523));
#95251=CARTESIAN_POINT('Ctrl Pts',(-3.02855730304457,2.92307692307692,-0.746474906977022));
#95252=CARTESIAN_POINT('Ctrl Pts',(-3.02885773675456,3.07692307692307,0.746548640155207));
#95253=CARTESIAN_POINT('Ctrl Pts',(-2.33474201794243,3.23076923076923,2.0684045486807));
#95254=CARTESIAN_POINT('Ctrl Pts',(-1.10621475336255,3.38461538461538,2.91679593290564));
#95255=CARTESIAN_POINT('Ctrl Pts',(0.376021898059204,3.53846153846154,3.09643080035079));
#95256=CARTESIAN_POINT('Ctrl Pts',(1.77197968324866,3.69230769230769,2.56735208320081));
#95257=CARTESIAN_POINT('Ctrl Pts',(2.76209532949166,3.84615384615385,1.44946426164245));
#95258=CARTESIAN_POINT('Ctrl Pts',(3.,3.94871794871795,0.483321946706125));
#95259=CARTESIAN_POINT('Ctrl Pts',(3.,4.,1.46957615897682E-15));
#95260=CARTESIAN_POINT('Origin',(2.5,4.,1.22464679914735E-15));
#95261=CARTESIAN_POINT('Origin',(2.5,4.,1.22464679914735E-15));
#95262=CARTESIAN_POINT('Origin',(2.5,7.2280144832367E-18,0.));
#99505=UNCERTAINTY_MEASURE_WITH_UNIT(LENGTH_MEASURE(0.01),#99527,
'DISTANCE_ACCURACY_VALUE',
'Maximum model space distance between geometric entities at asserted c
onnectivities');
#99508=UNCERTAINTY_MEASURE_WITH_UNIT(LENGTH_MEASURE(0.01),#99527,
'DISTANCE_ACCURACY_VALUE',
'Maximum model space distance between geometric entities at asserted c
onnectivities');
#99523=(
GEOMETRIC_REPRESENTATION_CONTEXT(3)
GLOBAL_UNCERTAINTY_ASSIGNED_CONTEXT((#99505))
GLOBAL_UNIT_ASSIGNED_CONTEXT((#99527,#99529,#99530))
REPRESENTATION_CONTEXT('','3D')
);
#99526=(
GEOMETRIC_REPRESENTATION_CONTEXT(3)
GLOBAL_UNCERTAINTY_ASSIGNED_CONTEXT((#99508))
GLOBAL_UNIT_ASSIGNED_CONTEXT((#99527,#99529,#99530))
REPRESENTATION_CONTEXT('','3D')
);
#99527=(
LENGTH_UNIT()
NAMED_UNIT(*)
SI_UNIT(.MILLI.,.METRE.)
);
#99529=(
NAMED_UNIT(*)
PLANE_ANGLE_UNIT()
SI_UNIT($,.RADIAN.)
);
#99530=(
NAMED_UNIT(*)
SI_UNIT($,.STERADIAN.)
SOLID_ANGLE_UNIT()
);
#99545=SHAPE_DEFINITION_REPRESENTATION(#99562,#99638);
#99562=PRODUCT_DEFINITION_SHAPE('',$,#99656);
#99638=SHAPE_REPRESENTATION('',(#19642),#99523);
#99641=PRODUCT_DEFINITION_CONTEXT('part definition',#99694,'design');
#99656=PRODUCT_DEFINITION('Compression spring','Compression spring',#99673,
#99641);
#99673=PRODUCT_DEFINITION_FORMATION('',$,#99710);
#99694=APPLICATION_CONTEXT(
'Core Data for Automotive Mechanical Design Process');
#99695=PRODUCT_CONTEXT('part definition',#99694,'mechanical');
#99710=PRODUCT('Compression spring','Compression spring',
'Reusable native Coil compression spring created and edited through Fu
sion UI. Mean diameter6mm, round wire1mm,2turns, overall free height5m
m; plain open ends. Axis+Y, initial wire centerY0, physical boundsY\X2\2212\X0\0.
5..4.5mm. Native parameters retain wire section when configuring worki
ng height4mm. No nonuniform body scaling or Boolean construction. Mate
rial temper, seats, stiffness, preload, buckling, fatigue and life not
 rated.',(#99695));
#99724=PRESENTATION_STYLE_ASSIGNMENT((#99737));
#99737=SURFACE_STYLE_USAGE(.BOTH.,#99750);
#99750=SURFACE_SIDE_STYLE('',(#99763));
#99763=SURFACE_STYLE_FILL_AREA(#99776);
#99776=FILL_AREA_STYLE('Spring gray',(#99789));
#99789=FILL_AREA_STYLE_COLOUR('Spring gray',#99802);
#99802=COLOUR_RGB('Spring gray',0.407843137254902,0.447058823529412,0.498039215686275);
ENDSEC;
END-ISO-10303-21;
